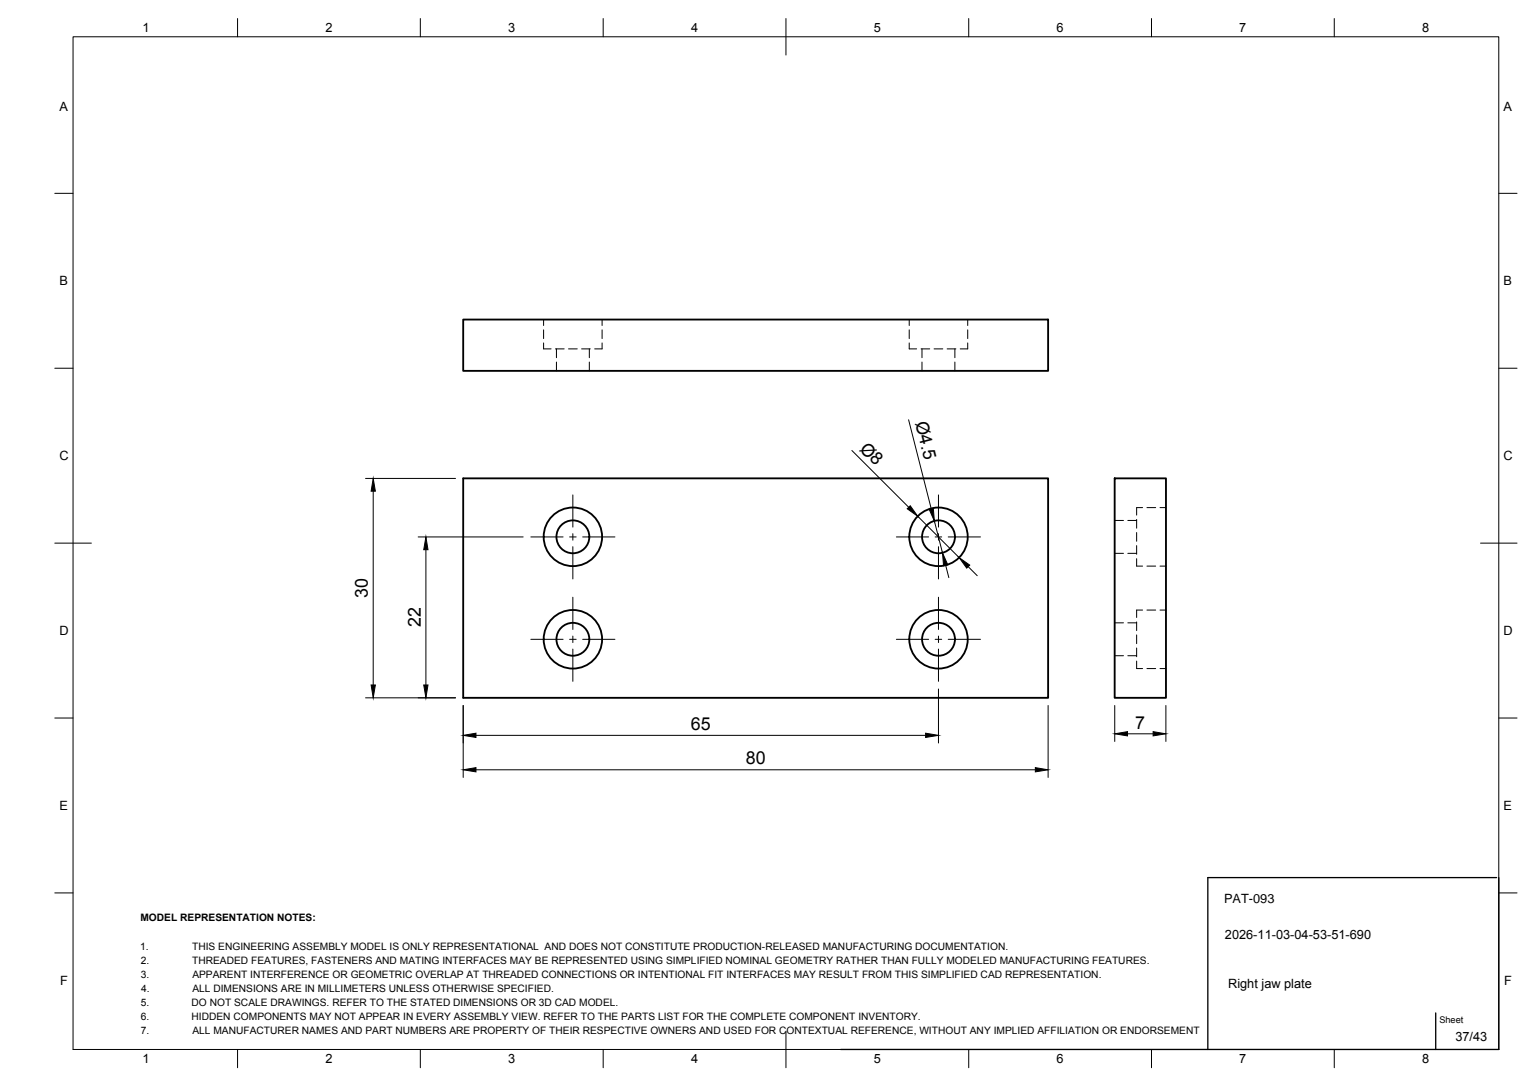
ISO-10303-21;
HEADER;
/* Generated by software containing ST-Developer
 * from STEP Tools, Inc. (www.steptools.com) 
 */

FILE_DESCRIPTION(
/* description */ ('Self-centering screw clamp'),
/* implementation_level */ '2;1');

FILE_NAME(
/* name */ 'Right jaw plate.step',
/* time_stamp */ '2026-10-28T03:25:31-07:00',
/* author */ (''),
/* organization */ (''),
/* preprocessor_version */ 'ST-DEVELOPER v20.2',
/* originating_system */ 'Autodesk Translation Framework v15.17.0.0',
/* authorisation */ '');

FILE_SCHEMA (('AUTOMOTIVE_DESIGN { 1 0 10303 214 3 1 1 }'));
ENDSEC;

DATA;
#10=MECHANICAL_DESIGN_GEOMETRIC_PRESENTATION_REPRESENTATION('',(#659),#16799);
#570=SHAPE_REPRESENTATION_RELATIONSHIP('SRR','None',#17046,#611);
#611=ADVANCED_BREP_SHAPE_REPRESENTATION('',(#707),#16784);
#659=STYLED_ITEM('',(#17319),#707);
#707=MANIFOLD_SOLID_BREP('Body1',#9110);
#969=FACE_BOUND('',#2399,.T.);
#970=FACE_BOUND('',#2402,.T.);
#971=FACE_BOUND('',#2405,.T.);
#972=FACE_BOUND('',#2408,.T.);
#973=FACE_BOUND('',#2415,.T.);
#974=FACE_BOUND('',#2416,.T.);
#975=FACE_BOUND('',#2417,.T.);
#976=FACE_BOUND('',#2418,.T.);
#977=FACE_BOUND('',#2421,.T.);
#978=FACE_BOUND('',#2422,.T.);
#979=FACE_BOUND('',#2423,.T.);
#980=FACE_BOUND('',#2424,.T.);
#1190=PLANE('',#10397);
#1191=PLANE('',#10402);
#1192=PLANE('',#10407);
#1193=PLANE('',#10412);
#1194=PLANE('',#10422);
#1195=PLANE('',#10423);
#1196=PLANE('',#10424);
#1197=PLANE('',#10425);
#1198=PLANE('',#10426);
#1199=PLANE('',#10427);
#1642=FACE_OUTER_BOUND('',#2397,.T.);
#1643=FACE_OUTER_BOUND('',#2398,.T.);
#1644=FACE_OUTER_BOUND('',#2400,.T.);
#1645=FACE_OUTER_BOUND('',#2401,.T.);
#1646=FACE_OUTER_BOUND('',#2403,.T.);
#1647=FACE_OUTER_BOUND('',#2404,.T.);
#1648=FACE_OUTER_BOUND('',#2406,.T.);
#1649=FACE_OUTER_BOUND('',#2407,.T.);
#1650=FACE_OUTER_BOUND('',#2409,.T.);
#1651=FACE_OUTER_BOUND('',#2410,.T.);
#1652=FACE_OUTER_BOUND('',#2411,.T.);
#1653=FACE_OUTER_BOUND('',#2412,.T.);
#1654=FACE_OUTER_BOUND('',#2413,.T.);
#1655=FACE_OUTER_BOUND('',#2414,.T.);
#1656=FACE_OUTER_BOUND('',#2419,.T.);
#1657=FACE_OUTER_BOUND('',#2420,.T.);
#1658=FACE_OUTER_BOUND('',#2425,.T.);
#1659=FACE_OUTER_BOUND('',#2426,.T.);
#2397=EDGE_LOOP('',(#7839,#7840,#7841,#7842));
#2398=EDGE_LOOP('',(#7843));
#2399=EDGE_LOOP('',(#7844));
#2400=EDGE_LOOP('',(#7845,#7846,#7847,#7848));
#2401=EDGE_LOOP('',(#7849));
#2402=EDGE_LOOP('',(#7850));
#2403=EDGE_LOOP('',(#7851,#7852,#7853,#7854));
#2404=EDGE_LOOP('',(#7855));
#2405=EDGE_LOOP('',(#7856));
#2406=EDGE_LOOP('',(#7857,#7858,#7859,#7860));
#2407=EDGE_LOOP('',(#7861));
#2408=EDGE_LOOP('',(#7862));
#2409=EDGE_LOOP('',(#7863,#7864,#7865,#7866));
#2410=EDGE_LOOP('',(#7867,#7868,#7869,#7870));
#2411=EDGE_LOOP('',(#7871,#7872,#7873,#7874));
#2412=EDGE_LOOP('',(#7875,#7876,#7877,#7878));
#2413=EDGE_LOOP('',(#7879,#7880,#7881,#7882));
#2414=EDGE_LOOP('',(#7883,#7884,#7885,#7886));
#2415=EDGE_LOOP('',(#7887));
#2416=EDGE_LOOP('',(#7888));
#2417=EDGE_LOOP('',(#7889));
#2418=EDGE_LOOP('',(#7890));
#2419=EDGE_LOOP('',(#7891,#7892,#7893,#7894));
#2420=EDGE_LOOP('',(#7895,#7896,#7897,#7898));
#2421=EDGE_LOOP('',(#7899));
#2422=EDGE_LOOP('',(#7900));
#2423=EDGE_LOOP('',(#7901));
#2424=EDGE_LOOP('',(#7902));
#2425=EDGE_LOOP('',(#7903,#7904,#7905,#7906));
#2426=EDGE_LOOP('',(#7907,#7908,#7909,#7910));
#3006=LINE('',#15903,#3579);
#3007=LINE('',#15912,#3580);
#3008=LINE('',#15921,#3581);
#3009=LINE('',#15930,#3582);
#3010=LINE('',#15937,#3583);
#3011=LINE('',#15941,#3584);
#3012=LINE('',#15945,#3585);
#3013=LINE('',#15949,#3586);
#3014=LINE('',#15954,#3587);
#3015=LINE('',#15956,#3588);
#3016=LINE('',#15958,#3589);
#3017=LINE('',#15959,#3590);
#3018=LINE('',#15962,#3591);
#3019=LINE('',#15964,#3592);
#3020=LINE('',#15965,#3593);
#3021=LINE('',#15968,#3594);
#3022=LINE('',#15970,#3595);
#3023=LINE('',#15971,#3596);
#3024=LINE('',#15973,#3597);
#3025=LINE('',#15974,#3598);
#3579=VECTOR('',#12819,0.4);
#3580=VECTOR('',#12830,0.4);
#3581=VECTOR('',#12841,0.4);
#3582=VECTOR('',#12852,0.4);
#3583=VECTOR('',#12861,0.225);
#3584=VECTOR('',#12866,0.225);
#3585=VECTOR('',#12871,0.225);
#3586=VECTOR('',#12876,0.225);
#3587=VECTOR('',#12881,1.);
#3588=VECTOR('',#12882,1.);
#3589=VECTOR('',#12883,1.);
#3590=VECTOR('',#12884,1.);
#3591=VECTOR('',#12887,1.);
#3592=VECTOR('',#12888,1.);
#3593=VECTOR('',#12889,1.);
#3594=VECTOR('',#12892,1.);
#3595=VECTOR('',#12893,1.);
#3596=VECTOR('',#12894,1.);
#3597=VECTOR('',#12897,1.);
#3598=VECTOR('',#12898,1.);
#4132=CIRCLE('',#10395,0.4);
#4133=CIRCLE('',#10396,0.4);
#4134=CIRCLE('',#10398,0.225);
#4135=CIRCLE('',#10400,0.4);
#4136=CIRCLE('',#10401,0.4);
#4137=CIRCLE('',#10403,0.225);
#4138=CIRCLE('',#10405,0.4);
#4139=CIRCLE('',#10406,0.4);
#4140=CIRCLE('',#10408,0.225);
#4141=CIRCLE('',#10410,0.4);
#4142=CIRCLE('',#10411,0.4);
#4143=CIRCLE('',#10413,0.225);
#4144=CIRCLE('',#10415,0.225);
#4145=CIRCLE('',#10417,0.225);
#4146=CIRCLE('',#10419,0.225);
#4147=CIRCLE('',#10421,0.225);
#4807=VERTEX_POINT('',#15900);
#4808=VERTEX_POINT('',#15902);
#4809=VERTEX_POINT('',#15906);
#4810=VERTEX_POINT('',#15909);
#4811=VERTEX_POINT('',#15911);
#4812=VERTEX_POINT('',#15915);
#4813=VERTEX_POINT('',#15918);
#4814=VERTEX_POINT('',#15920);
#4815=VERTEX_POINT('',#15924);
#4816=VERTEX_POINT('',#15927);
#4817=VERTEX_POINT('',#15929);
#4818=VERTEX_POINT('',#15933);
#4819=VERTEX_POINT('',#15936);
#4820=VERTEX_POINT('',#15940);
#4821=VERTEX_POINT('',#15944);
#4822=VERTEX_POINT('',#15948);
#4823=VERTEX_POINT('',#15952);
#4824=VERTEX_POINT('',#15953);
#4825=VERTEX_POINT('',#15955);
#4826=VERTEX_POINT('',#15957);
#4827=VERTEX_POINT('',#15961);
#4828=VERTEX_POINT('',#15963);
#4829=VERTEX_POINT('',#15967);
#4830=VERTEX_POINT('',#15969);
#5844=EDGE_CURVE('',#4807,#4807,#4132,.T.);
#5845=EDGE_CURVE('',#4807,#4808,#3006,.T.);
#5846=EDGE_CURVE('',#4808,#4808,#4133,.T.);
#5847=EDGE_CURVE('',#4809,#4809,#4134,.T.);
#5848=EDGE_CURVE('',#4810,#4810,#4135,.T.);
#5849=EDGE_CURVE('',#4810,#4811,#3007,.T.);
#5850=EDGE_CURVE('',#4811,#4811,#4136,.T.);
#5851=EDGE_CURVE('',#4812,#4812,#4137,.T.);
#5852=EDGE_CURVE('',#4813,#4813,#4138,.T.);
#5853=EDGE_CURVE('',#4813,#4814,#3008,.T.);
#5854=EDGE_CURVE('',#4814,#4814,#4139,.T.);
#5855=EDGE_CURVE('',#4815,#4815,#4140,.T.);
#5856=EDGE_CURVE('',#4816,#4816,#4141,.T.);
#5857=EDGE_CURVE('',#4816,#4817,#3009,.T.);
#5858=EDGE_CURVE('',#4817,#4817,#4142,.T.);
#5859=EDGE_CURVE('',#4818,#4818,#4143,.T.);
#5860=EDGE_CURVE('',#4809,#4819,#3010,.T.);
#5861=EDGE_CURVE('',#4819,#4819,#4144,.T.);
#5862=EDGE_CURVE('',#4812,#4820,#3011,.T.);
#5863=EDGE_CURVE('',#4820,#4820,#4145,.T.);
#5864=EDGE_CURVE('',#4815,#4821,#3012,.T.);
#5865=EDGE_CURVE('',#4821,#4821,#4146,.T.);
#5866=EDGE_CURVE('',#4818,#4822,#3013,.T.);
#5867=EDGE_CURVE('',#4822,#4822,#4147,.T.);
#5868=EDGE_CURVE('',#4823,#4824,#3014,.T.);
#5869=EDGE_CURVE('',#4824,#4825,#3015,.T.);
#5870=EDGE_CURVE('',#4826,#4825,#3016,.T.);
#5871=EDGE_CURVE('',#4823,#4826,#3017,.T.);
#5872=EDGE_CURVE('',#4827,#4823,#3018,.T.);
#5873=EDGE_CURVE('',#4828,#4826,#3019,.T.);
#5874=EDGE_CURVE('',#4827,#4828,#3020,.T.);
#5875=EDGE_CURVE('',#4829,#4827,#3021,.T.);
#5876=EDGE_CURVE('',#4830,#4828,#3022,.T.);
#5877=EDGE_CURVE('',#4829,#4830,#3023,.T.);
#5878=EDGE_CURVE('',#4824,#4829,#3024,.T.);
#5879=EDGE_CURVE('',#4825,#4830,#3025,.T.);
#7839=ORIENTED_EDGE('',*,*,#5844,.F.);
#7840=ORIENTED_EDGE('',*,*,#5845,.T.);
#7841=ORIENTED_EDGE('',*,*,#5846,.T.);
#7842=ORIENTED_EDGE('',*,*,#5845,.F.);
#7843=ORIENTED_EDGE('',*,*,#5846,.F.);
#7844=ORIENTED_EDGE('',*,*,#5847,.F.);
#7845=ORIENTED_EDGE('',*,*,#5848,.F.);
#7846=ORIENTED_EDGE('',*,*,#5849,.T.);
#7847=ORIENTED_EDGE('',*,*,#5850,.T.);
#7848=ORIENTED_EDGE('',*,*,#5849,.F.);
#7849=ORIENTED_EDGE('',*,*,#5850,.F.);
#7850=ORIENTED_EDGE('',*,*,#5851,.F.);
#7851=ORIENTED_EDGE('',*,*,#5852,.F.);
#7852=ORIENTED_EDGE('',*,*,#5853,.T.);
#7853=ORIENTED_EDGE('',*,*,#5854,.T.);
#7854=ORIENTED_EDGE('',*,*,#5853,.F.);
#7855=ORIENTED_EDGE('',*,*,#5854,.F.);
#7856=ORIENTED_EDGE('',*,*,#5855,.F.);
#7857=ORIENTED_EDGE('',*,*,#5856,.F.);
#7858=ORIENTED_EDGE('',*,*,#5857,.T.);
#7859=ORIENTED_EDGE('',*,*,#5858,.T.);
#7860=ORIENTED_EDGE('',*,*,#5857,.F.);
#7861=ORIENTED_EDGE('',*,*,#5858,.F.);
#7862=ORIENTED_EDGE('',*,*,#5859,.F.);
#7863=ORIENTED_EDGE('',*,*,#5847,.T.);
#7864=ORIENTED_EDGE('',*,*,#5860,.T.);
#7865=ORIENTED_EDGE('',*,*,#5861,.F.);
#7866=ORIENTED_EDGE('',*,*,#5860,.F.);
#7867=ORIENTED_EDGE('',*,*,#5851,.T.);
#7868=ORIENTED_EDGE('',*,*,#5862,.T.);
#7869=ORIENTED_EDGE('',*,*,#5863,.F.);
#7870=ORIENTED_EDGE('',*,*,#5862,.F.);
#7871=ORIENTED_EDGE('',*,*,#5855,.T.);
#7872=ORIENTED_EDGE('',*,*,#5864,.T.);
#7873=ORIENTED_EDGE('',*,*,#5865,.F.);
#7874=ORIENTED_EDGE('',*,*,#5864,.F.);
#7875=ORIENTED_EDGE('',*,*,#5859,.T.);
#7876=ORIENTED_EDGE('',*,*,#5866,.T.);
#7877=ORIENTED_EDGE('',*,*,#5867,.F.);
#7878=ORIENTED_EDGE('',*,*,#5866,.F.);
#7879=ORIENTED_EDGE('',*,*,#5868,.T.);
#7880=ORIENTED_EDGE('',*,*,#5869,.T.);
#7881=ORIENTED_EDGE('',*,*,#5870,.F.);
#7882=ORIENTED_EDGE('',*,*,#5871,.F.);
#7883=ORIENTED_EDGE('',*,*,#5872,.T.);
#7884=ORIENTED_EDGE('',*,*,#5871,.T.);
#7885=ORIENTED_EDGE('',*,*,#5873,.F.);
#7886=ORIENTED_EDGE('',*,*,#5874,.F.);
#7887=ORIENTED_EDGE('',*,*,#5861,.T.);
#7888=ORIENTED_EDGE('',*,*,#5863,.T.);
#7889=ORIENTED_EDGE('',*,*,#5865,.T.);
#7890=ORIENTED_EDGE('',*,*,#5867,.T.);
#7891=ORIENTED_EDGE('',*,*,#5875,.T.);
#7892=ORIENTED_EDGE('',*,*,#5874,.T.);
#7893=ORIENTED_EDGE('',*,*,#5876,.F.);
#7894=ORIENTED_EDGE('',*,*,#5877,.F.);
#7895=ORIENTED_EDGE('',*,*,#5878,.T.);
#7896=ORIENTED_EDGE('',*,*,#5877,.T.);
#7897=ORIENTED_EDGE('',*,*,#5879,.F.);
#7898=ORIENTED_EDGE('',*,*,#5869,.F.);
#7899=ORIENTED_EDGE('',*,*,#5856,.T.);
#7900=ORIENTED_EDGE('',*,*,#5852,.T.);
#7901=ORIENTED_EDGE('',*,*,#5848,.T.);
#7902=ORIENTED_EDGE('',*,*,#5844,.T.);
#7903=ORIENTED_EDGE('',*,*,#5879,.T.);
#7904=ORIENTED_EDGE('',*,*,#5876,.T.);
#7905=ORIENTED_EDGE('',*,*,#5873,.T.);
#7906=ORIENTED_EDGE('',*,*,#5870,.T.);
#7907=ORIENTED_EDGE('',*,*,#5878,.F.);
#7908=ORIENTED_EDGE('',*,*,#5868,.F.);
#7909=ORIENTED_EDGE('',*,*,#5872,.F.);
#7910=ORIENTED_EDGE('',*,*,#5875,.F.);
#8528=CYLINDRICAL_SURFACE('',#10394,0.4);
#8529=CYLINDRICAL_SURFACE('',#10399,0.4);
#8530=CYLINDRICAL_SURFACE('',#10404,0.4);
#8531=CYLINDRICAL_SURFACE('',#10409,0.4);
#8532=CYLINDRICAL_SURFACE('',#10414,0.225);
#8533=CYLINDRICAL_SURFACE('',#10416,0.225);
#8534=CYLINDRICAL_SURFACE('',#10418,0.225);
#8535=CYLINDRICAL_SURFACE('',#10420,0.225);
#8940=ADVANCED_FACE('',(#1642),#8528,.F.);
#8941=ADVANCED_FACE('',(#1643,#969),#1190,.F.);
#8942=ADVANCED_FACE('',(#1644),#8529,.F.);
#8943=ADVANCED_FACE('',(#1645,#970),#1191,.F.);
#8944=ADVANCED_FACE('',(#1646),#8530,.F.);
#8945=ADVANCED_FACE('',(#1647,#971),#1192,.F.);
#8946=ADVANCED_FACE('',(#1648),#8531,.F.);
#8947=ADVANCED_FACE('',(#1649,#972),#1193,.F.);
#8948=ADVANCED_FACE('',(#1650),#8532,.F.);
#8949=ADVANCED_FACE('',(#1651),#8533,.F.);
#8950=ADVANCED_FACE('',(#1652),#8534,.F.);
#8951=ADVANCED_FACE('',(#1653),#8535,.F.);
#8952=ADVANCED_FACE('',(#1654),#1194,.T.);
#8953=ADVANCED_FACE('',(#1655,#973,#974,#975,#976),#1195,.T.);
#8954=ADVANCED_FACE('',(#1656),#1196,.T.);
#8955=ADVANCED_FACE('',(#1657,#977,#978,#979,#980),#1197,.T.);
#8956=ADVANCED_FACE('',(#1658),#1198,.T.);
#8957=ADVANCED_FACE('',(#1659),#1199,.F.);
#9110=CLOSED_SHELL('',(#8940,#8941,#8942,#8943,#8944,#8945,#8946,#8947,
#8948,#8949,#8950,#8951,#8952,#8953,#8954,#8955,#8956,#8957));
#10393=AXIS2_PLACEMENT_3D('',#15898,#12813,#12814);
#10394=AXIS2_PLACEMENT_3D('',#15899,#12815,#12816);
#10395=AXIS2_PLACEMENT_3D('',#15901,#12817,#12818);
#10396=AXIS2_PLACEMENT_3D('',#15904,#12820,#12821);
#10397=AXIS2_PLACEMENT_3D('',#15905,#12822,#12823);
#10398=AXIS2_PLACEMENT_3D('',#15907,#12824,#12825);
#10399=AXIS2_PLACEMENT_3D('',#15908,#12826,#12827);
#10400=AXIS2_PLACEMENT_3D('',#15910,#12828,#12829);
#10401=AXIS2_PLACEMENT_3D('',#15913,#12831,#12832);
#10402=AXIS2_PLACEMENT_3D('',#15914,#12833,#12834);
#10403=AXIS2_PLACEMENT_3D('',#15916,#12835,#12836);
#10404=AXIS2_PLACEMENT_3D('',#15917,#12837,#12838);
#10405=AXIS2_PLACEMENT_3D('',#15919,#12839,#12840);
#10406=AXIS2_PLACEMENT_3D('',#15922,#12842,#12843);
#10407=AXIS2_PLACEMENT_3D('',#15923,#12844,#12845);
#10408=AXIS2_PLACEMENT_3D('',#15925,#12846,#12847);
#10409=AXIS2_PLACEMENT_3D('',#15926,#12848,#12849);
#10410=AXIS2_PLACEMENT_3D('',#15928,#12850,#12851);
#10411=AXIS2_PLACEMENT_3D('',#15931,#12853,#12854);
#10412=AXIS2_PLACEMENT_3D('',#15932,#12855,#12856);
#10413=AXIS2_PLACEMENT_3D('',#15934,#12857,#12858);
#10414=AXIS2_PLACEMENT_3D('',#15935,#12859,#12860);
#10415=AXIS2_PLACEMENT_3D('',#15938,#12862,#12863);
#10416=AXIS2_PLACEMENT_3D('',#15939,#12864,#12865);
#10417=AXIS2_PLACEMENT_3D('',#15942,#12867,#12868);
#10418=AXIS2_PLACEMENT_3D('',#15943,#12869,#12870);
#10419=AXIS2_PLACEMENT_3D('',#15946,#12872,#12873);
#10420=AXIS2_PLACEMENT_3D('',#15947,#12874,#12875);
#10421=AXIS2_PLACEMENT_3D('',#15950,#12877,#12878);
#10422=AXIS2_PLACEMENT_3D('',#15951,#12879,#12880);
#10423=AXIS2_PLACEMENT_3D('',#15960,#12885,#12886);
#10424=AXIS2_PLACEMENT_3D('',#15966,#12890,#12891);
#10425=AXIS2_PLACEMENT_3D('',#15972,#12895,#12896);
#10426=AXIS2_PLACEMENT_3D('',#15975,#12899,#12900);
#10427=AXIS2_PLACEMENT_3D('',#15976,#12901,#12902);
#12813=DIRECTION('axis',(0.,0.,1.));
#12814=DIRECTION('refdir',(1.,0.,0.));
#12815=DIRECTION('center_axis',(1.,0.,0.));
#12816=DIRECTION('ref_axis',(0.,0.,-1.));
#12817=DIRECTION('center_axis',(1.,0.,0.));
#12818=DIRECTION('ref_axis',(0.,0.,-1.));
#12819=DIRECTION('',(1.,0.,0.));
#12820=DIRECTION('center_axis',(1.,0.,0.));
#12821=DIRECTION('ref_axis',(0.,0.,-1.));
#12822=DIRECTION('center_axis',(1.,0.,0.));
#12823=DIRECTION('ref_axis',(0.,0.,-1.));
#12824=DIRECTION('center_axis',(-1.,0.,0.));
#12825=DIRECTION('ref_axis',(0.,0.,-1.));
#12826=DIRECTION('center_axis',(1.,0.,0.));
#12827=DIRECTION('ref_axis',(0.,0.,-1.));
#12828=DIRECTION('center_axis',(1.,0.,0.));
#12829=DIRECTION('ref_axis',(0.,0.,-1.));
#12830=DIRECTION('',(1.,0.,0.));
#12831=DIRECTION('center_axis',(1.,0.,0.));
#12832=DIRECTION('ref_axis',(0.,0.,-1.));
#12833=DIRECTION('center_axis',(1.,0.,0.));
#12834=DIRECTION('ref_axis',(0.,0.,-1.));
#12835=DIRECTION('center_axis',(-1.,0.,0.));
#12836=DIRECTION('ref_axis',(0.,0.,-1.));
#12837=DIRECTION('center_axis',(1.,0.,0.));
#12838=DIRECTION('ref_axis',(0.,0.,-1.));
#12839=DIRECTION('center_axis',(1.,0.,0.));
#12840=DIRECTION('ref_axis',(0.,0.,-1.));
#12841=DIRECTION('',(1.,0.,0.));
#12842=DIRECTION('center_axis',(1.,0.,0.));
#12843=DIRECTION('ref_axis',(0.,0.,-1.));
#12844=DIRECTION('center_axis',(1.,0.,0.));
#12845=DIRECTION('ref_axis',(0.,0.,-1.));
#12846=DIRECTION('center_axis',(-1.,0.,0.));
#12847=DIRECTION('ref_axis',(0.,0.,-1.));
#12848=DIRECTION('center_axis',(1.,0.,0.));
#12849=DIRECTION('ref_axis',(0.,0.,-1.));
#12850=DIRECTION('center_axis',(1.,0.,0.));
#12851=DIRECTION('ref_axis',(0.,0.,-1.));
#12852=DIRECTION('',(1.,0.,0.));
#12853=DIRECTION('center_axis',(1.,0.,0.));
#12854=DIRECTION('ref_axis',(0.,0.,-1.));
#12855=DIRECTION('center_axis',(1.,0.,0.));
#12856=DIRECTION('ref_axis',(0.,0.,-1.));
#12857=DIRECTION('center_axis',(-1.,0.,0.));
#12858=DIRECTION('ref_axis',(0.,0.,-1.));
#12859=DIRECTION('center_axis',(1.,0.,0.));
#12860=DIRECTION('ref_axis',(0.,0.,-1.));
#12861=DIRECTION('',(1.,0.,0.));
#12862=DIRECTION('center_axis',(-1.,0.,0.));
#12863=DIRECTION('ref_axis',(0.,0.,-1.));
#12864=DIRECTION('center_axis',(1.,0.,0.));
#12865=DIRECTION('ref_axis',(0.,0.,-1.));
#12866=DIRECTION('',(1.,0.,0.));
#12867=DIRECTION('center_axis',(-1.,0.,0.));
#12868=DIRECTION('ref_axis',(0.,0.,-1.));
#12869=DIRECTION('center_axis',(1.,0.,0.));
#12870=DIRECTION('ref_axis',(0.,0.,-1.));
#12871=DIRECTION('',(1.,0.,0.));
#12872=DIRECTION('center_axis',(-1.,0.,0.));
#12873=DIRECTION('ref_axis',(0.,0.,-1.));
#12874=DIRECTION('center_axis',(1.,0.,0.));
#12875=DIRECTION('ref_axis',(0.,0.,-1.));
#12876=DIRECTION('',(1.,0.,0.));
#12877=DIRECTION('center_axis',(-1.,0.,0.));
#12878=DIRECTION('ref_axis',(0.,0.,-1.));
#12879=DIRECTION('center_axis',(0.,1.,0.));
#12880=DIRECTION('ref_axis',(-1.,0.,0.));
#12881=DIRECTION('',(-1.,0.,0.));
#12882=DIRECTION('',(0.,0.,1.));
#12883=DIRECTION('',(-1.,0.,0.));
#12884=DIRECTION('',(0.,0.,1.));
#12885=DIRECTION('center_axis',(1.,0.,0.));
#12886=DIRECTION('ref_axis',(0.,1.,0.));
#12887=DIRECTION('',(0.,1.,0.));
#12888=DIRECTION('',(0.,1.,0.));
#12889=DIRECTION('',(0.,0.,1.));
#12890=DIRECTION('center_axis',(0.,-1.,0.));
#12891=DIRECTION('ref_axis',(1.,0.,0.));
#12892=DIRECTION('',(1.,0.,0.));
#12893=DIRECTION('',(1.,0.,0.));
#12894=DIRECTION('',(0.,0.,1.));
#12895=DIRECTION('center_axis',(-1.,0.,0.));
#12896=DIRECTION('ref_axis',(0.,-1.,0.));
#12897=DIRECTION('',(0.,-1.,0.));
#12898=DIRECTION('',(0.,-1.,0.));
#12899=DIRECTION('center_axis',(0.,0.,1.));
#12900=DIRECTION('ref_axis',(1.,0.,0.));
#12901=DIRECTION('center_axis',(0.,0.,1.));
#12902=DIRECTION('ref_axis',(1.,0.,0.));
#15898=CARTESIAN_POINT('',(0.,0.,0.));
#15899=CARTESIAN_POINT('Origin',(4.7,2.5,7.8));
#15900=CARTESIAN_POINT('',(4.8,2.5,8.2));
#15901=CARTESIAN_POINT('Origin',(4.8,2.5,7.8));
#15902=CARTESIAN_POINT('',(5.2,2.5,8.2));
#15903=CARTESIAN_POINT('',(4.7,2.5,8.2));
#15904=CARTESIAN_POINT('Origin',(5.2,2.5,7.8));
#15905=CARTESIAN_POINT('Origin',(5.2,2.5,7.8));
#15906=CARTESIAN_POINT('',(5.2,2.5,8.025));
#15907=CARTESIAN_POINT('Origin',(5.2,2.5,7.8));
#15908=CARTESIAN_POINT('Origin',(4.7,-2.5,9.2));
#15909=CARTESIAN_POINT('',(4.8,-2.5,9.6));
#15910=CARTESIAN_POINT('Origin',(4.8,-2.5,9.2));
#15911=CARTESIAN_POINT('',(5.2,-2.5,9.6));
#15912=CARTESIAN_POINT('',(4.7,-2.5,9.6));
#15913=CARTESIAN_POINT('Origin',(5.2,-2.5,9.2));
#15914=CARTESIAN_POINT('Origin',(5.2,-2.5,9.2));
#15915=CARTESIAN_POINT('',(5.2,-2.5,9.425));
#15916=CARTESIAN_POINT('Origin',(5.2,-2.5,9.2));
#15917=CARTESIAN_POINT('Origin',(4.7,-2.5,7.8));
#15918=CARTESIAN_POINT('',(4.8,-2.5,8.2));
#15919=CARTESIAN_POINT('Origin',(4.8,-2.5,7.8));
#15920=CARTESIAN_POINT('',(5.2,-2.5,8.2));
#15921=CARTESIAN_POINT('',(4.7,-2.5,8.2));
#15922=CARTESIAN_POINT('Origin',(5.2,-2.5,7.8));
#15923=CARTESIAN_POINT('Origin',(5.2,-2.5,7.8));
#15924=CARTESIAN_POINT('',(5.2,-2.5,8.025));
#15925=CARTESIAN_POINT('Origin',(5.2,-2.5,7.8));
#15926=CARTESIAN_POINT('Origin',(4.7,2.5,9.2));
#15927=CARTESIAN_POINT('',(4.8,2.5,9.6));
#15928=CARTESIAN_POINT('Origin',(4.8,2.5,9.2));
#15929=CARTESIAN_POINT('',(5.2,2.5,9.6));
#15930=CARTESIAN_POINT('',(4.7,2.5,9.6));
#15931=CARTESIAN_POINT('Origin',(5.2,2.5,9.2));
#15932=CARTESIAN_POINT('Origin',(5.2,2.5,9.2));
#15933=CARTESIAN_POINT('',(5.2,2.5,9.425));
#15934=CARTESIAN_POINT('Origin',(5.2,2.5,9.2));
#15935=CARTESIAN_POINT('Origin',(4.7,2.5,7.8));
#15936=CARTESIAN_POINT('',(5.5,2.5,8.025));
#15937=CARTESIAN_POINT('',(4.7,2.5,8.025));
#15938=CARTESIAN_POINT('Origin',(5.5,2.5,7.8));
#15939=CARTESIAN_POINT('Origin',(4.7,-2.5,9.2));
#15940=CARTESIAN_POINT('',(5.5,-2.5,9.425));
#15941=CARTESIAN_POINT('',(4.7,-2.5,9.425));
#15942=CARTESIAN_POINT('Origin',(5.5,-2.5,9.2));
#15943=CARTESIAN_POINT('Origin',(4.7,-2.5,7.8));
#15944=CARTESIAN_POINT('',(5.5,-2.5,8.025));
#15945=CARTESIAN_POINT('',(4.7,-2.5,8.025));
#15946=CARTESIAN_POINT('Origin',(5.5,-2.5,7.8));
#15947=CARTESIAN_POINT('Origin',(4.7,2.5,9.2));
#15948=CARTESIAN_POINT('',(5.5,2.5,9.425));
#15949=CARTESIAN_POINT('',(4.7,2.5,9.425));
#15950=CARTESIAN_POINT('Origin',(5.5,2.5,9.2));
#15951=CARTESIAN_POINT('Origin',(5.5,4.,7.));
#15952=CARTESIAN_POINT('',(5.5,4.,7.));
#15953=CARTESIAN_POINT('',(4.8,4.,7.));
#15954=CARTESIAN_POINT('',(5.5,4.,7.));
#15955=CARTESIAN_POINT('',(4.8,4.,10.));
#15956=CARTESIAN_POINT('',(4.8,4.,7.));
#15957=CARTESIAN_POINT('',(5.5,4.,10.));
#15958=CARTESIAN_POINT('',(5.5,4.,10.));
#15959=CARTESIAN_POINT('',(5.5,4.,7.));
#15960=CARTESIAN_POINT('Origin',(5.5,-4.,7.));
#15961=CARTESIAN_POINT('',(5.5,-4.,7.));
#15962=CARTESIAN_POINT('',(5.5,-4.,7.));
#15963=CARTESIAN_POINT('',(5.5,-4.,10.));
#15964=CARTESIAN_POINT('',(5.5,-4.,10.));
#15965=CARTESIAN_POINT('',(5.5,-4.,7.));
#15966=CARTESIAN_POINT('Origin',(4.8,-4.,7.));
#15967=CARTESIAN_POINT('',(4.8,-4.,7.));
#15968=CARTESIAN_POINT('',(4.8,-4.,7.));
#15969=CARTESIAN_POINT('',(4.8,-4.,10.));
#15970=CARTESIAN_POINT('',(4.8,-4.,10.));
#15971=CARTESIAN_POINT('',(4.8,-4.,7.));
#15972=CARTESIAN_POINT('Origin',(4.8,4.,7.));
#15973=CARTESIAN_POINT('',(4.8,4.,7.));
#15974=CARTESIAN_POINT('',(4.8,4.,10.));
#15975=CARTESIAN_POINT('Origin',(5.15,0.,10.));
#15976=CARTESIAN_POINT('Origin',(5.15,0.,7.));
#16735=UNCERTAINTY_MEASURE_WITH_UNIT(LENGTH_MEASURE(0.001),#16800,
'DISTANCE_ACCURACY_VALUE',
'Maximum model space distance between geometric entities at asserted c
onnectivities');
#16750=UNCERTAINTY_MEASURE_WITH_UNIT(LENGTH_MEASURE(0.001),#16800,
'DISTANCE_ACCURACY_VALUE',
'Maximum model space distance between geometric entities at asserted c
onnectivities');
#16784=(
GEOMETRIC_REPRESENTATION_CONTEXT(3)
GLOBAL_UNCERTAINTY_ASSIGNED_CONTEXT((#16735))
GLOBAL_UNIT_ASSIGNED_CONTEXT((#16800,#16802,#16803))
REPRESENTATION_CONTEXT('','3D')
);
#16799=(
GEOMETRIC_REPRESENTATION_CONTEXT(3)
GLOBAL_UNCERTAINTY_ASSIGNED_CONTEXT((#16750))
GLOBAL_UNIT_ASSIGNED_CONTEXT((#16800,#16802,#16803))
REPRESENTATION_CONTEXT('','3D')
);
#16800=(
LENGTH_UNIT()
NAMED_UNIT(*)
SI_UNIT(.CENTI.,.METRE.)
);
#16802=(
NAMED_UNIT(*)
PLANE_ANGLE_UNIT()
SI_UNIT($,.RADIAN.)
);
#16803=(
NAMED_UNIT(*)
SI_UNIT($,.STERADIAN.)
SOLID_ANGLE_UNIT()
);
#16837=SHAPE_DEFINITION_REPRESENTATION(#16890,#17046);
#16890=PRODUCT_DEFINITION_SHAPE('',$,#17095);
#17046=SHAPE_REPRESENTATION('',(#10393),#16784);
#17061=PRODUCT_DEFINITION_CONTEXT('part definition',#17207,'design');
#17095=PRODUCT_DEFINITION('Right jaw plate','Right jaw plate',#17143,#17061);
#17143=PRODUCT_DEFINITION_FORMATION('',$,#17242);
#17207=APPLICATION_CONTEXT(
'Core Data for Automotive Mechanical Design Process');
#17208=PRODUCT_CONTEXT('part definition',#17207,'mechanical');
#17242=PRODUCT('Right jaw plate','Right jaw plate','Right jaw plate',(#17208));
#17313=COLOUR_RGB('Sky Blue',0.24,0.69,0.87);
#17314=FILL_AREA_STYLE_COLOUR('',#17313);
#17315=FILL_AREA_STYLE('',(#17314));
#17316=SURFACE_STYLE_FILL_AREA(#17315);
#17317=SURFACE_SIDE_STYLE('',(#17316));
#17318=SURFACE_STYLE_USAGE(.BOTH.,#17317);
#17319=PRESENTATION_STYLE_ASSIGNMENT((#17318));
ENDSEC;
END-ISO-10303-21;
